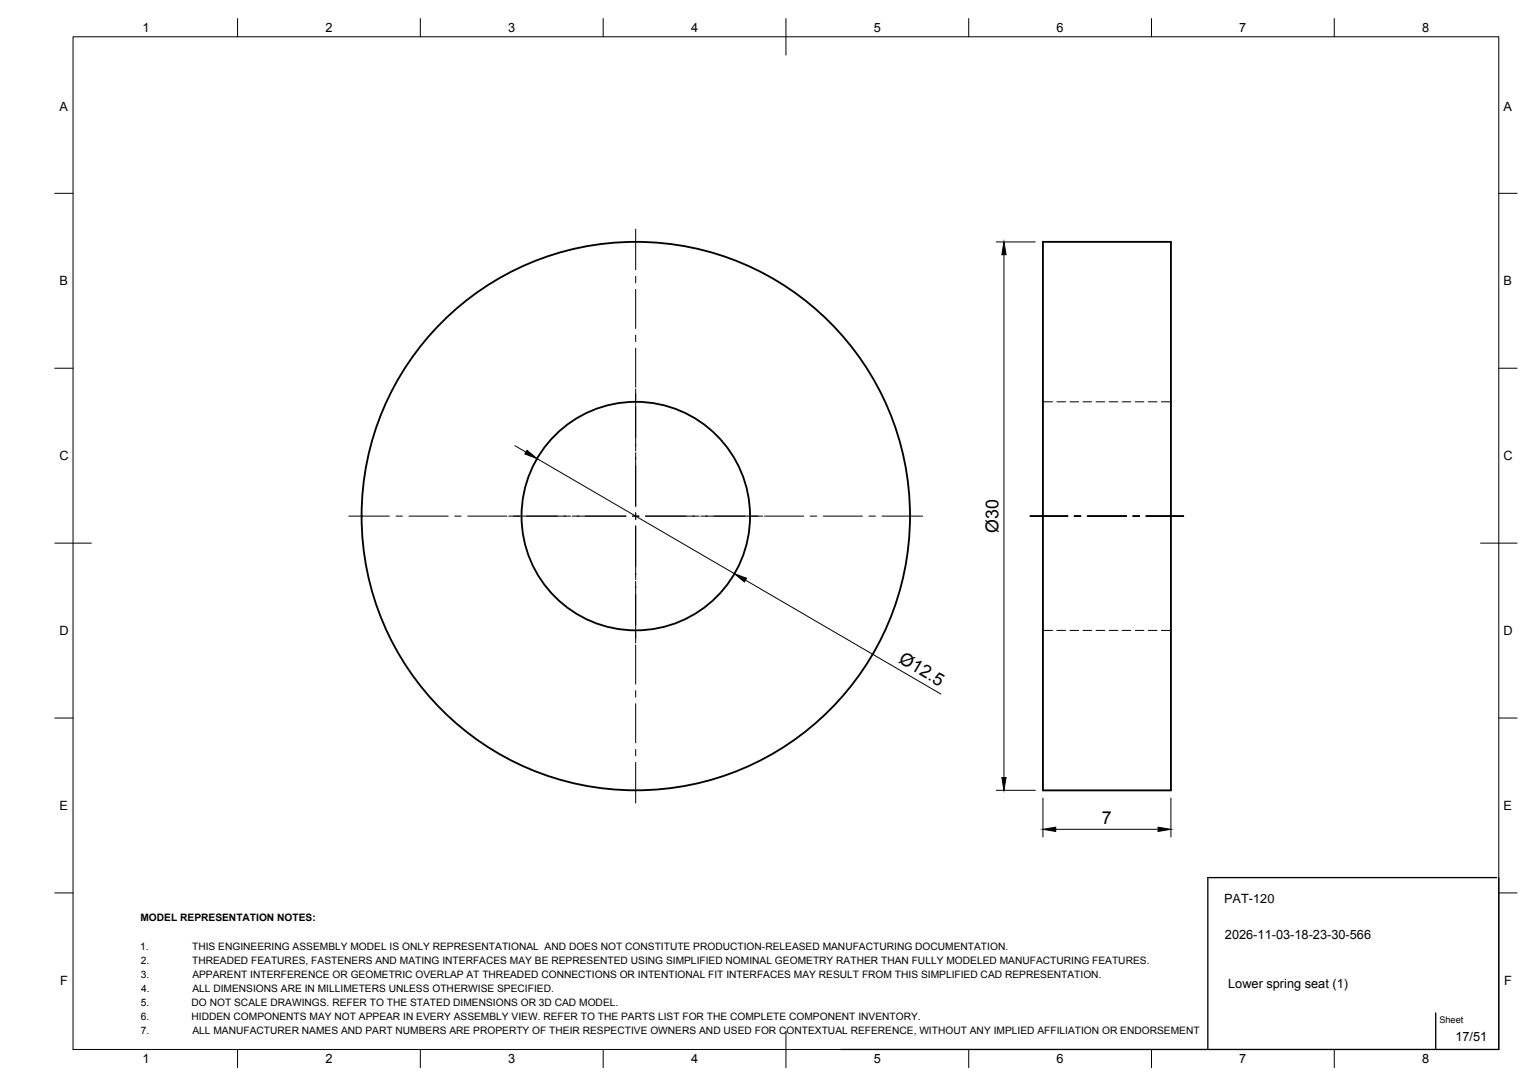
ISO-10303-21;
HEADER;
/* Generated by software containing ST-Developer
 * from STEP Tools, Inc. (www.steptools.com) 
 */

FILE_DESCRIPTION(
/* description */ ('Vibration shaker table dummy'),
/* implementation_level */ '2;1');

FILE_NAME(
/* name */ 'Lower spring seat (1).step',
/* time_stamp */ '2026-10-27T10:55:14-07:00',
/* author */ (''),
/* organization */ (''),
/* preprocessor_version */ 'ST-DEVELOPER v20.2',
/* originating_system */ 'Autodesk Translation Framework v15.17.0.0',
/* authorisation */ '');

FILE_SCHEMA (('AUTOMOTIVE_DESIGN { 1 0 10303 214 3 1 1 }'));
ENDSEC;

DATA;
#10=MECHANICAL_DESIGN_GEOMETRIC_PRESENTATION_REPRESENTATION('',(#698),#22394);
#606=SHAPE_REPRESENTATION_RELATIONSHIP('SRR','None',#22652,#652);
#652=ADVANCED_BREP_SHAPE_REPRESENTATION('',(#744),#22358);
#698=STYLED_ITEM('',(#22961),#744);
#744=MANIFOLD_SOLID_BREP('Body1',#9216);
#889=FACE_BOUND('',#2107,.T.);
#890=FACE_BOUND('',#2109,.T.);
#1144=PLANE('',#10073);
#1145=PLANE('',#10074);
#1492=FACE_OUTER_BOUND('',#2104,.T.);
#1493=FACE_OUTER_BOUND('',#2105,.T.);
#1494=FACE_OUTER_BOUND('',#2106,.T.);
#1495=FACE_OUTER_BOUND('',#2108,.T.);
#2104=EDGE_LOOP('',(#6960,#6961,#6962,#6963));
#2105=EDGE_LOOP('',(#6964,#6965,#6966,#6967));
#2106=EDGE_LOOP('',(#6968));
#2107=EDGE_LOOP('',(#6969));
#2108=EDGE_LOOP('',(#6970));
#2109=EDGE_LOOP('',(#6971));
#2836=LINE('',#16186,#3455);
#2837=LINE('',#16192,#3456);
#3455=VECTOR('',#11782,0.625);
#3456=VECTOR('',#11789,1.5);
#4002=CIRCLE('',#10068,0.625);
#4003=CIRCLE('',#10069,0.625);
#4004=CIRCLE('',#10071,1.5);
#4005=CIRCLE('',#10072,1.5);
#4605=VERTEX_POINT('',#16183);
#4606=VERTEX_POINT('',#16185);
#4607=VERTEX_POINT('',#16189);
#4608=VERTEX_POINT('',#16191);
#5473=EDGE_CURVE('',#4605,#4605,#4002,.T.);
#5474=EDGE_CURVE('',#4605,#4606,#2836,.T.);
#5475=EDGE_CURVE('',#4606,#4606,#4003,.T.);
#5476=EDGE_CURVE('',#4607,#4607,#4004,.T.);
#5477=EDGE_CURVE('',#4607,#4608,#2837,.T.);
#5478=EDGE_CURVE('',#4608,#4608,#4005,.T.);
#6960=ORIENTED_EDGE('',*,*,#5473,.F.);
#6961=ORIENTED_EDGE('',*,*,#5474,.T.);
#6962=ORIENTED_EDGE('',*,*,#5475,.T.);
#6963=ORIENTED_EDGE('',*,*,#5474,.F.);
#6964=ORIENTED_EDGE('',*,*,#5476,.F.);
#6965=ORIENTED_EDGE('',*,*,#5477,.T.);
#6966=ORIENTED_EDGE('',*,*,#5478,.T.);
#6967=ORIENTED_EDGE('',*,*,#5477,.F.);
#6968=ORIENTED_EDGE('',*,*,#5476,.T.);
#6969=ORIENTED_EDGE('',*,*,#5473,.T.);
#6970=ORIENTED_EDGE('',*,*,#5478,.F.);
#6971=ORIENTED_EDGE('',*,*,#5475,.F.);
#8572=CYLINDRICAL_SURFACE('',#10067,0.625);
#8573=CYLINDRICAL_SURFACE('',#10070,1.5);
#8857=ADVANCED_FACE('',(#1492),#8572,.F.);
#8858=ADVANCED_FACE('',(#1493),#8573,.T.);
#8859=ADVANCED_FACE('',(#1494,#889),#1144,.T.);
#8860=ADVANCED_FACE('',(#1495,#890),#1145,.F.);
#9216=CLOSED_SHELL('',(#8857,#8858,#8859,#8860));
#10066=AXIS2_PLACEMENT_3D('',#16181,#11776,#11777);
#10067=AXIS2_PLACEMENT_3D('',#16182,#11778,#11779);
#10068=AXIS2_PLACEMENT_3D('',#16184,#11780,#11781);
#10069=AXIS2_PLACEMENT_3D('',#16187,#11783,#11784);
#10070=AXIS2_PLACEMENT_3D('',#16188,#11785,#11786);
#10071=AXIS2_PLACEMENT_3D('',#16190,#11787,#11788);
#10072=AXIS2_PLACEMENT_3D('',#16193,#11790,#11791);
#10073=AXIS2_PLACEMENT_3D('',#16194,#11792,#11793);
#10074=AXIS2_PLACEMENT_3D('',#16195,#11794,#11795);
#11776=DIRECTION('axis',(0.,0.,1.));
#11777=DIRECTION('refdir',(1.,0.,0.));
#11778=DIRECTION('center_axis',(0.,0.,1.));
#11779=DIRECTION('ref_axis',(1.,0.,0.));
#11780=DIRECTION('center_axis',(0.,0.,-1.));
#11781=DIRECTION('ref_axis',(1.,0.,0.));
#11782=DIRECTION('',(0.,0.,-1.));
#11783=DIRECTION('center_axis',(0.,0.,-1.));
#11784=DIRECTION('ref_axis',(1.,0.,0.));
#11785=DIRECTION('center_axis',(0.,0.,1.));
#11786=DIRECTION('ref_axis',(1.,0.,0.));
#11787=DIRECTION('center_axis',(0.,0.,1.));
#11788=DIRECTION('ref_axis',(1.,0.,0.));
#11789=DIRECTION('',(0.,0.,-1.));
#11790=DIRECTION('center_axis',(0.,0.,1.));
#11791=DIRECTION('ref_axis',(1.,0.,0.));
#11792=DIRECTION('center_axis',(0.,0.,1.));
#11793=DIRECTION('ref_axis',(1.,0.,0.));
#11794=DIRECTION('center_axis',(0.,0.,1.));
#11795=DIRECTION('ref_axis',(1.,0.,0.));
#16181=CARTESIAN_POINT('',(0.,0.,0.));
#16182=CARTESIAN_POINT('Origin',(-6.,4.,1.9));
#16183=CARTESIAN_POINT('',(-6.625,4.,2.6));
#16184=CARTESIAN_POINT('Origin',(-6.,4.,2.6));
#16185=CARTESIAN_POINT('',(-6.625,4.,1.9));
#16186=CARTESIAN_POINT('',(-6.625,4.,1.9));
#16187=CARTESIAN_POINT('Origin',(-6.,4.,1.9));
#16188=CARTESIAN_POINT('Origin',(-6.,4.,1.9));
#16189=CARTESIAN_POINT('',(-7.5,4.,2.6));
#16190=CARTESIAN_POINT('Origin',(-6.,4.,2.6));
#16191=CARTESIAN_POINT('',(-7.5,4.,1.9));
#16192=CARTESIAN_POINT('',(-7.5,4.,1.9));
#16193=CARTESIAN_POINT('Origin',(-6.,4.,1.9));
#16194=CARTESIAN_POINT('Origin',(-6.,4.,2.6));
#16195=CARTESIAN_POINT('Origin',(-6.,4.,1.9));
#22307=UNCERTAINTY_MEASURE_WITH_UNIT(LENGTH_MEASURE(0.001),#22395,
'DISTANCE_ACCURACY_VALUE',
'Maximum model space distance between geometric entities at asserted c
onnectivities');
#22343=UNCERTAINTY_MEASURE_WITH_UNIT(LENGTH_MEASURE(0.001),#22395,
'DISTANCE_ACCURACY_VALUE',
'Maximum model space distance between geometric entities at asserted c
onnectivities');
#22358=(
GEOMETRIC_REPRESENTATION_CONTEXT(3)
GLOBAL_UNCERTAINTY_ASSIGNED_CONTEXT((#22307))
GLOBAL_UNIT_ASSIGNED_CONTEXT((#22395,#22397,#22398))
REPRESENTATION_CONTEXT('','3D')
);
#22394=(
GEOMETRIC_REPRESENTATION_CONTEXT(3)
GLOBAL_UNCERTAINTY_ASSIGNED_CONTEXT((#22343))
GLOBAL_UNIT_ASSIGNED_CONTEXT((#22395,#22397,#22398))
REPRESENTATION_CONTEXT('','3D')
);
#22395=(
LENGTH_UNIT()
NAMED_UNIT(*)
SI_UNIT(.CENTI.,.METRE.)
);
#22397=(
NAMED_UNIT(*)
PLANE_ANGLE_UNIT()
SI_UNIT($,.RADIAN.)
);
#22398=(
NAMED_UNIT(*)
SI_UNIT($,.STERADIAN.)
SOLID_ANGLE_UNIT()
);
#22413=SHAPE_DEFINITION_REPRESENTATION(#22463,#22652);
#22463=PRODUCT_DEFINITION_SHAPE('',$,#22703);
#22652=SHAPE_REPRESENTATION('',(#10066),#22358);
#22688=PRODUCT_DEFINITION_CONTEXT('part definition',#22840,'design');
#22703=PRODUCT_DEFINITION('Lower spring seat (1)','Lower spring seat (1)',
#22753,#22688);
#22753=PRODUCT_DEFINITION_FORMATION('',$,#22856);
#22840=APPLICATION_CONTEXT(
'Core Data for Automotive Mechanical Design Process');
#22841=PRODUCT_CONTEXT('part definition',#22840,'mechanical');
#22856=PRODUCT('Lower spring seat (1)','Lower spring seat (1)',
'Lower spring seat (1)',(#22841));
#22955=COLOUR_RGB('Grey',0.48,0.52,0.57);
#22956=FILL_AREA_STYLE_COLOUR('',#22955);
#22957=FILL_AREA_STYLE('',(#22956));
#22958=SURFACE_STYLE_FILL_AREA(#22957);
#22959=SURFACE_SIDE_STYLE('',(#22958));
#22960=SURFACE_STYLE_USAGE(.BOTH.,#22959);
#22961=PRESENTATION_STYLE_ASSIGNMENT((#22960));
ENDSEC;
END-ISO-10303-21;
